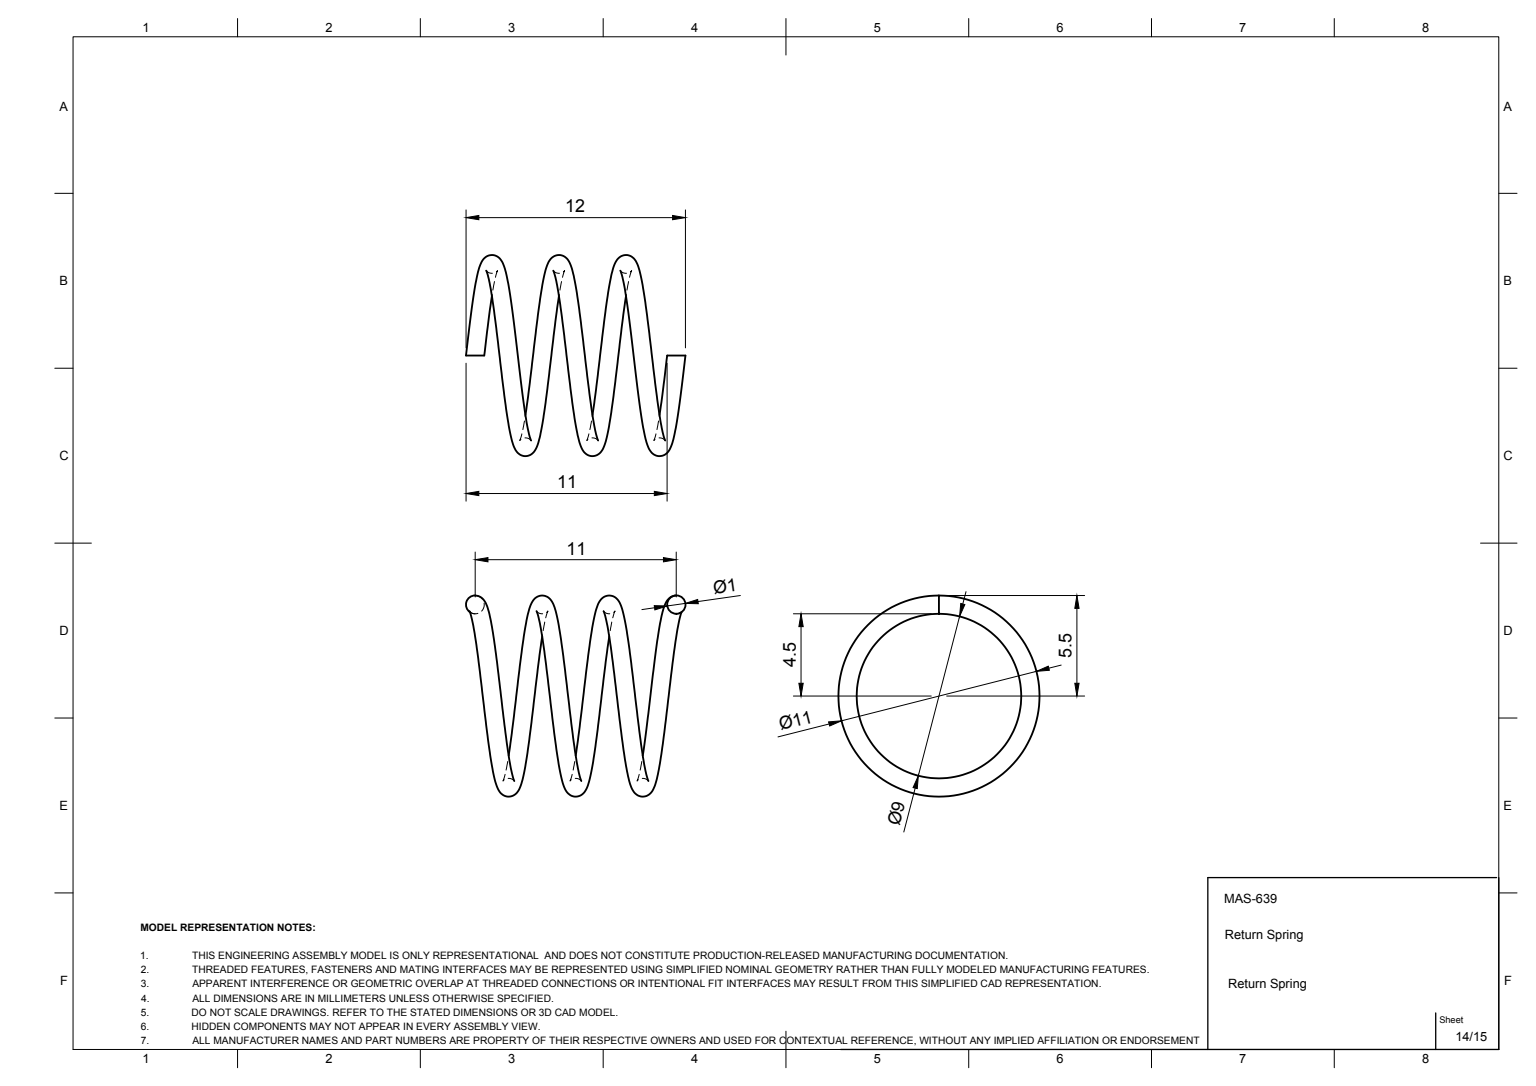
ISO-10303-21;
HEADER;
/* Generated by software containing ST-Developer
 * from STEP Tools, Inc. (www.steptools.com) 
 */

FILE_DESCRIPTION(
/* description */ ('Independent maintained push-to-latch/pull-to-reset mushroom-operator 
CAD. Two opposed spring-loaded ball detents in turned circular seats b
ias both travel stops; direct normally-closed bridge opens6mm when pre
ssed. Rounded palm/pull rim, captured head screw, removable detent clo
sures, native Coil spring families, insulated shared terminals and ord
inary machining features. Manual geometric states and ideal same-mater
ial spring-energy direction only; no electrical/safety certification, 
force/contact dynamics, wear, load or life rating. Requested blue/gray
 visual palette, not safety identification. External wiring/anchors an
d application engineering omitted.'),
/* implementation_level */ '2;1');

FILE_NAME(
/* name */ 'Return spring.step',
/* time_stamp */ '2026-11-08T17:54:26-08:00',
/* author */ (''),
/* organization */ (''),
/* preprocessor_version */ 'ST-DEVELOPER v20.2',
/* originating_system */ 'Autodesk Translation Framework v15.17.0.0',
/* authorisation */ '');

FILE_SCHEMA (('AUTOMOTIVE_DESIGN { 1 0 10303 214 3 1 1 }'));
ENDSEC;

DATA;
#10=MECHANICAL_DESIGN_GEOMETRIC_PRESENTATION_REPRESENTATION('',(#196),#43980);
#162=SHAPE_REPRESENTATION_RELATIONSHIP('SRR','None',#44062,#179);
#179=ADVANCED_BREP_SHAPE_REPRESENTATION('',(#213),#43969);
#196=STYLED_ITEM('',(#44155),#213);
#213=MANIFOLD_SOLID_BREP('Body1',#11237);
#242=B_SPLINE_SURFACE_WITH_KNOTS('',3,3,((#29398,#29399,#29400,#29401,#29402,
#29403,#29404,#29405,#29406,#29407,#29408,#29409,#29410,#29411,#29412,#29413,
#29414,#29415,#29416,#29417,#29418,#29419,#29420,#29421,#29422,#29423,#29424,
#29425,#29426,#29427,#29428,#29429,#29430,#29431,#29432,#29433,#29434,#29435,
#29436,#29437,#29438),(#29439,#29440,#29441,#29442,#29443,#29444,#29445,
#29446,#29447,#29448,#29449,#29450,#29451,#29452,#29453,#29454,#29455,#29456,
#29457,#29458,#29459,#29460,#29461,#29462,#29463,#29464,#29465,#29466,#29467,
#29468,#29469,#29470,#29471,#29472,#29473,#29474,#29475,#29476,#29477,#29478,
#29479),(#29480,#29481,#29482,#29483,#29484,#29485,#29486,#29487,#29488,
#29489,#29490,#29491,#29492,#29493,#29494,#29495,#29496,#29497,#29498,#29499,
#29500,#29501,#29502,#29503,#29504,#29505,#29506,#29507,#29508,#29509,#29510,
#29511,#29512,#29513,#29514,#29515,#29516,#29517,#29518,#29519,#29520),
(#29521,#29522,#29523,#29524,#29525,#29526,#29527,#29528,#29529,#29530,
#29531,#29532,#29533,#29534,#29535,#29536,#29537,#29538,#29539,#29540,#29541,
#29542,#29543,#29544,#29545,#29546,#29547,#29548,#29549,#29550,#29551,#29552,
#29553,#29554,#29555,#29556,#29557,#29558,#29559,#29560,#29561),(#29562,
#29563,#29564,#29565,#29566,#29567,#29568,#29569,#29570,#29571,#29572,#29573,
#29574,#29575,#29576,#29577,#29578,#29579,#29580,#29581,#29582,#29583,#29584,
#29585,#29586,#29587,#29588,#29589,#29590,#29591,#29592,#29593,#29594,#29595,
#29596,#29597,#29598,#29599,#29600,#29601,#29602),(#29603,#29604,#29605,
#29606,#29607,#29608,#29609,#29610,#29611,#29612,#29613,#29614,#29615,#29616,
#29617,#29618,#29619,#29620,#29621,#29622,#29623,#29624,#29625,#29626,#29627,
#29628,#29629,#29630,#29631,#29632,#29633,#29634,#29635,#29636,#29637,#29638,
#29639,#29640,#29641,#29642,#29643),(#29644,#29645,#29646,#29647,#29648,
#29649,#29650,#29651,#29652,#29653,#29654,#29655,#29656,#29657,#29658,#29659,
#29660,#29661,#29662,#29663,#29664,#29665,#29666,#29667,#29668,#29669,#29670,
#29671,#29672,#29673,#29674,#29675,#29676,#29677,#29678,#29679,#29680,#29681,
#29682,#29683,#29684),(#29685,#29686,#29687,#29688,#29689,#29690,#29691,
#29692,#29693,#29694,#29695,#29696,#29697,#29698,#29699,#29700,#29701,#29702,
#29703,#29704,#29705,#29706,#29707,#29708,#29709,#29710,#29711,#29712,#29713,
#29714,#29715,#29716,#29717,#29718,#29719,#29720,#29721,#29722,#29723,#29724,
#29725),(#29726,#29727,#29728,#29729,#29730,#29731,#29732,#29733,#29734,
#29735,#29736,#29737,#29738,#29739,#29740,#29741,#29742,#29743,#29744,#29745,
#29746,#29747,#29748,#29749,#29750,#29751,#29752,#29753,#29754,#29755,#29756,
#29757,#29758,#29759,#29760,#29761,#29762,#29763,#29764,#29765,#29766),
(#29767,#29768,#29769,#29770,#29771,#29772,#29773,#29774,#29775,#29776,
#29777,#29778,#29779,#29780,#29781,#29782,#29783,#29784,#29785,#29786,#29787,
#29788,#29789,#29790,#29791,#29792,#29793,#29794,#29795,#29796,#29797,#29798,
#29799,#29800,#29801,#29802,#29803,#29804,#29805,#29806,#29807)),
 .UNSPECIFIED.,.T.,.F.,.F.,(4,1,1,1,1,1,1,4),(4,1,1,1,1,1,1,1,1,1,1,1,1,
1,1,1,1,1,1,1,1,1,1,1,1,1,1,1,1,1,1,1,1,1,1,1,1,1,4),(-3.14159265358979,
-2.24399475256414,-1.34639685153848,-0.448798950512828,0.448798950512828,
1.34639685153848,2.24399475256414,3.14159265358979),(0.,0.496040945303652,
0.992081890607303,1.48812283591095,1.98416378121461,2.48020472651826,2.97624567182191,
3.47228661712556,3.96832756242921,4.46436850773286,4.96040945303652,5.45645039834017,
5.95249134364382,6.44853228894747,6.94457323425112,7.44061417955477,7.93665512485842,
8.43269607016208,8.92873701546573,9.42477796076938,9.92081890607303,10.4168598513767,
10.9129007966803,11.408941741984,11.9049826872876,12.4010236325913,12.8970645778949,
13.3931055231986,13.8891464685022,14.3851874138059,14.8812283591095,15.3772693044132,
15.8733102497168,16.3693511950205,16.8653921403242,17.3614330856278,17.8574740309315,
18.3535149762351,18.8495559215388),.UNSPECIFIED.);
#411=PLANE('',#11894);
#412=PLANE('',#11895);
#817=FACE_OUTER_BOUND('',#1496,.T.);
#818=FACE_OUTER_BOUND('',#1497,.T.);
#819=FACE_OUTER_BOUND('',#1498,.T.);
#1496=EDGE_LOOP('',(#8645,#8646,#8647,#8648));
#1497=EDGE_LOOP('',(#8649));
#1498=EDGE_LOOP('',(#8650));
#1934=CIRCLE('',#11892,0.05);
#1935=CIRCLE('',#11893,0.05);
#2421=B_SPLINE_CURVE_WITH_KNOTS('',3,(#29811,#29812,#29813,#29814,#29815,
#29816,#29817,#29818,#29819,#29820,#29821,#29822,#29823,#29824,#29825,#29826,
#29827,#29828,#29829,#29830,#29831,#29832,#29833,#29834,#29835,#29836,#29837,
#29838,#29839,#29840,#29841,#29842,#29843,#29844,#29845,#29846,#29847,#29848,
#29849,#29850,#29851),.UNSPECIFIED.,.F.,.F.,(4,1,1,1,1,1,1,1,1,1,1,1,1,
1,1,1,1,1,1,1,1,1,1,1,1,1,1,1,1,1,1,1,1,1,1,1,1,1,4),(0.,0.496040945303652,
0.992081890607303,1.48812283591095,1.98416378121461,2.48020472651826,2.97624567182191,
3.47228661712556,3.96832756242921,4.46436850773286,4.96040945303652,5.45645039834017,
5.95249134364382,6.44853228894747,6.94457323425112,7.44061417955477,7.93665512485842,
8.43269607016208,8.92873701546573,9.42477796076938,9.92081890607303,10.4168598513767,
10.9129007966803,11.408941741984,11.9049826872876,12.4010236325913,12.8970645778949,
13.3931055231986,13.8891464685022,14.3851874138059,14.8812283591095,15.3772693044132,
15.8733102497168,16.3693511950205,16.8653921403242,17.3614330856278,17.8574740309315,
18.3535149762351,18.8495559215388),.UNSPECIFIED.);
#4686=VERTEX_POINT('',#29808);
#4687=VERTEX_POINT('',#29810);
#6092=EDGE_CURVE('',#4686,#4686,#1934,.T.);
#6093=EDGE_CURVE('',#4686,#4687,#2421,.T.);
#6094=EDGE_CURVE('',#4687,#4687,#1935,.T.);
#8645=ORIENTED_EDGE('',*,*,#6092,.T.);
#8646=ORIENTED_EDGE('',*,*,#6093,.T.);
#8647=ORIENTED_EDGE('',*,*,#6094,.F.);
#8648=ORIENTED_EDGE('',*,*,#6093,.F.);
#8649=ORIENTED_EDGE('',*,*,#6094,.T.);
#8650=ORIENTED_EDGE('',*,*,#6092,.F.);
#10942=ADVANCED_FACE('',(#817),#242,.T.);
#10943=ADVANCED_FACE('',(#818),#411,.F.);
#10944=ADVANCED_FACE('',(#819),#412,.T.);
#11237=CLOSED_SHELL('',(#10942,#10943,#10944));
#11891=AXIS2_PLACEMENT_3D('',#29397,#13507,#13508);
#11892=AXIS2_PLACEMENT_3D('',#29809,#13509,#13510);
#11893=AXIS2_PLACEMENT_3D('',#29852,#13511,#13512);
#11894=AXIS2_PLACEMENT_3D('',#29853,#13513,#13514);
#11895=AXIS2_PLACEMENT_3D('',#29854,#13515,#13516);
#13507=DIRECTION('axis',(0.,0.,1.));
#13508=DIRECTION('refdir',(1.,0.,0.));
#13509=DIRECTION('center_axis',(0.,0.,-1.));
#13510=DIRECTION('ref_axis',(-1.,0.,0.));
#13511=DIRECTION('center_axis',(7.34788079488412E-16,0.,-1.));
#13512=DIRECTION('ref_axis',(-1.,0.,-7.34788079488412E-16));
#13513=DIRECTION('center_axis',(-7.34788079488412E-16,0.,1.));
#13514=DIRECTION('ref_axis',(1.,0.,7.34788079488412E-16));
#13515=DIRECTION('center_axis',(0.,0.,1.));
#13516=DIRECTION('ref_axis',(1.,0.,0.));
#29397=CARTESIAN_POINT('',(0.,0.,0.));
#29398=CARTESIAN_POINT('Ctrl Pts',(0.55,-6.12323399573676E-18,0.));
#29399=CARTESIAN_POINT('Ctrl Pts',(0.55,0.00964912280701754,-0.0909408399723361));
#29400=CARTESIAN_POINT('Ctrl Pts',(0.504021197632585,0.0289473684210526,
-0.272733075266705));
#29401=CARTESIAN_POINT('Ctrl Pts',(0.313429112214632,0.0578947368421053,
-0.4797633508545));
#29402=CARTESIAN_POINT('Ctrl Pts',(0.0473287281417178,0.0868421052631579,
-0.571108104224167));
#29403=CARTESIAN_POINT('Ctrl Pts',(-0.230201927212741,0.115789473684211,
-0.52480399893423));
#29404=CARTESIAN_POINT('Ctrl Pts',(-0.452231273974558,0.144736842105263,
-0.351985646771294));
#29405=CARTESIAN_POINT('Ctrl Pts',(-0.565254339124195,0.173684210526316,
-0.0943246722345097));
#29406=CARTESIAN_POINT('Ctrl Pts',(-0.542018875701069,0.202631578947368,
0.186075664943732));
#29407=CARTESIAN_POINT('Ctrl Pts',(-0.388129668188505,0.231578947368421,
0.421620932468086));
#29408=CARTESIAN_POINT('Ctrl Pts',(-0.140680214568305,0.260526315789474,
0.555533945989301));
#29409=CARTESIAN_POINT('Ctrl Pts',(0.140680250766997,0.289473684210526,
0.555533855939788));
#29410=CARTESIAN_POINT('Ctrl Pts',(0.388129540647023,0.318421052631579,
0.421621069647034));
#29411=CARTESIAN_POINT('Ctrl Pts',(0.542019161337126,0.347368421052632,
0.186075408839635));
#29412=CARTESIAN_POINT('Ctrl Pts',(0.565253745898005,0.376315789473684,
-0.0943241631669167));
#29413=CARTESIAN_POINT('Ctrl Pts',(0.452232485289668,0.405263157894737,
-0.351986675242114));
#29414=CARTESIAN_POINT('Ctrl Pts',(0.230199463455902,0.43421052631579,-0.524801912662064));
#29415=CARTESIAN_POINT('Ctrl Pts',(-0.0473237183527974,0.463157894736842,
-0.571112341965111));
#29416=CARTESIAN_POINT('Ctrl Pts',(-0.313439397484805,0.492105263157895,
-0.479754713047896));
#29417=CARTESIAN_POINT('Ctrl Pts',(-0.503999728127626,0.521052631578947,
-0.272751013161366));
#29418=CARTESIAN_POINT('Ctrl Pts',(-0.573069664876904,0.55,-2.39751545989516E-16));
#29419=CARTESIAN_POINT('Ctrl Pts',(-0.503999728127627,0.578947368421053,
0.272751013161366));
#29420=CARTESIAN_POINT('Ctrl Pts',(-0.313439397484805,0.607894736842105,
0.479754713047896));
#29421=CARTESIAN_POINT('Ctrl Pts',(-0.0473237183527982,0.636842105263158,
0.571112341965112));
#29422=CARTESIAN_POINT('Ctrl Pts',(0.230199463455903,0.665789473684211,
0.524801912662064));
#29423=CARTESIAN_POINT('Ctrl Pts',(0.452232485289667,0.694736842105263,
0.351986675242114));
#29424=CARTESIAN_POINT('Ctrl Pts',(0.565253745898007,0.723684210526316,
0.0943241631669169));
#29425=CARTESIAN_POINT('Ctrl Pts',(0.542019161337125,0.752631578947369,
-0.186075408839635));
#29426=CARTESIAN_POINT('Ctrl Pts',(0.388129540647024,0.781578947368421,
-0.421621069647034));
#29427=CARTESIAN_POINT('Ctrl Pts',(0.140680250766998,0.810526315789474,
-0.555533855939788));
#29428=CARTESIAN_POINT('Ctrl Pts',(-0.140680214568305,0.839473684210527,
-0.555533945989301));
#29429=CARTESIAN_POINT('Ctrl Pts',(-0.388129668188505,0.868421052631579,
-0.421620932468086));
#29430=CARTESIAN_POINT('Ctrl Pts',(-0.542018875701069,0.897368421052632,
-0.186075664943732));
#29431=CARTESIAN_POINT('Ctrl Pts',(-0.565254339124195,0.926315789473684,
0.0943246722345097));
#29432=CARTESIAN_POINT('Ctrl Pts',(-0.452231273974558,0.955263157894737,
0.351985646771295));
#29433=CARTESIAN_POINT('Ctrl Pts',(-0.23020192721274,0.984210526315789,
0.52480399893423));
#29434=CARTESIAN_POINT('Ctrl Pts',(0.047328728141718,1.01315789473684,0.571108104224167));
#29435=CARTESIAN_POINT('Ctrl Pts',(0.313429112214631,1.04210526315789,0.4797633508545));
#29436=CARTESIAN_POINT('Ctrl Pts',(0.504021197632586,1.07105263157895,0.272733075266706));
#29437=CARTESIAN_POINT('Ctrl Pts',(0.55,1.09035087719298,0.0909408399723365));
#29438=CARTESIAN_POINT('Ctrl Pts',(0.55,1.1,4.04133443718627E-16));
#29439=CARTESIAN_POINT('Ctrl Pts',(0.55,-0.0149599650170943,0.));
#29440=CARTESIAN_POINT('Ctrl Pts',(0.55,-0.0053108422100767,-0.090963337566431));
#29441=CARTESIAN_POINT('Ctrl Pts',(0.504025597995316,0.0139874034039583,
-0.272722100402085));
#29442=CARTESIAN_POINT('Ctrl Pts',(0.313430222123197,0.0429347718250111,
-0.479772059039409));
#29443=CARTESIAN_POINT('Ctrl Pts',(0.0473293473867347,0.0718821402460636,
-0.57110852263267));
#29444=CARTESIAN_POINT('Ctrl Pts',(-0.230203431837132,0.100829508667116,
-0.524808465895466));
#29445=CARTESIAN_POINT('Ctrl Pts',(-0.452233813118511,0.129776877088169,
-0.351986987289247));
#29446=CARTESIAN_POINT('Ctrl Pts',(-0.565257658331638,0.158724245509222,
-0.0943255642817947));
#29447=CARTESIAN_POINT('Ctrl Pts',(-0.54202199880764,0.187671613930274,
0.186076913937926));
#29448=CARTESIAN_POINT('Ctrl Pts',(-0.388131929047426,0.216618982351327,
0.421623293944921));
#29449=CARTESIAN_POINT('Ctrl Pts',(-0.140681025512686,0.245566350772379,
0.555537208898314));
#29450=CARTESIAN_POINT('Ctrl Pts',(0.140681064202504,0.274513719193432,
0.555537057388092));
#29451=CARTESIAN_POINT('Ctrl Pts',(0.388131792728783,0.303461087614485,
0.421623524751422));
#29452=CARTESIAN_POINT('Ctrl Pts',(0.542022304100625,0.332408456035537,
0.186076483037303));
#29453=CARTESIAN_POINT('Ctrl Pts',(0.565257024280752,0.36135582445659,-0.0943247077642448));
#29454=CARTESIAN_POINT('Ctrl Pts',(0.452235107794019,0.390303192877642,
-0.351988717720502));
#29455=CARTESIAN_POINT('Ctrl Pts',(0.230200798529239,0.419250561298696,
-0.524804955578026));
#29456=CARTESIAN_POINT('Ctrl Pts',(-0.0473239928336781,0.448197929719748,
-0.571115654320144));
#29457=CARTESIAN_POINT('Ctrl Pts',(-0.313441215206083,0.477145298140801,
-0.479757495171017));
#29458=CARTESIAN_POINT('Ctrl Pts',(-0.504002650999897,0.506092666561853,
-0.272752594988184));
#29459=CARTESIAN_POINT('Ctrl Pts',(-0.573072988290107,0.535040034982906,
-2.69720489238206E-16));
#29460=CARTESIAN_POINT('Ctrl Pts',(-0.504002650999898,0.563987403403958,
0.272752594988184));
#29461=CARTESIAN_POINT('Ctrl Pts',(-0.313441215206083,0.59293477182501,
0.479757495171017));
#29462=CARTESIAN_POINT('Ctrl Pts',(-0.0473239928336784,0.621882140246064,
0.571115654320144));
#29463=CARTESIAN_POINT('Ctrl Pts',(0.230200798529239,0.650829508667116,
0.524804955578026));
#29464=CARTESIAN_POINT('Ctrl Pts',(0.452235107794019,0.67977687708817,0.351988717720502));
#29465=CARTESIAN_POINT('Ctrl Pts',(0.565257024280752,0.708724245509221,
0.0943247077642448));
#29466=CARTESIAN_POINT('Ctrl Pts',(0.542022304100626,0.737671613930275,
-0.186076483037303));
#29467=CARTESIAN_POINT('Ctrl Pts',(0.388131792728783,0.766618982351327,
-0.421623524751422));
#29468=CARTESIAN_POINT('Ctrl Pts',(0.140681064202504,0.79556635077238,-0.555537057388092));
#29469=CARTESIAN_POINT('Ctrl Pts',(-0.140681025512686,0.824513719193432,
-0.555537208898314));
#29470=CARTESIAN_POINT('Ctrl Pts',(-0.388131929047426,0.853461087614485,
-0.421623293944921));
#29471=CARTESIAN_POINT('Ctrl Pts',(-0.54202199880764,0.882408456035538,
-0.186076913937926));
#29472=CARTESIAN_POINT('Ctrl Pts',(-0.565257658331638,0.911355824456589,
0.094325564281795));
#29473=CARTESIAN_POINT('Ctrl Pts',(-0.452233813118511,0.940303192877643,
0.351986987289247));
#29474=CARTESIAN_POINT('Ctrl Pts',(-0.230203431837132,0.969250561298695,
0.524808465895466));
#29475=CARTESIAN_POINT('Ctrl Pts',(0.0473293473867349,0.998197929719749,
0.57110852263267));
#29476=CARTESIAN_POINT('Ctrl Pts',(0.313430222123197,1.0271452981408,0.47977205903941));
#29477=CARTESIAN_POINT('Ctrl Pts',(0.504025597995316,1.05609266656185,0.272722100402085));
#29478=CARTESIAN_POINT('Ctrl Pts',(0.55,1.07539091217589,0.0909633375664313));
#29479=CARTESIAN_POINT('Ctrl Pts',(0.55,1.08504003498291,4.04133443718627E-16));
#29480=CARTESIAN_POINT('Ctrl Pts',(0.53570113931992,-0.0447553195607142,
0.));
#29481=CARTESIAN_POINT('Ctrl Pts',(0.53570113931992,-0.0351061967536967,
-0.0885671891766316));
#29482=CARTESIAN_POINT('Ctrl Pts',(0.490915856431254,-0.0158079511396616,
-0.265647154764381));
#29483=CARTESIAN_POINT('Ctrl Pts',(0.305280141935785,0.013139417281391,
-0.467286867853663));
#29484=CARTESIAN_POINT('Ctrl Pts',(0.0460980211403113,0.0420867857024435,
-0.556260302160471));
#29485=CARTESIAN_POINT('Ctrl Pts',(-0.224216526816036,0.0710341541234964,
-0.511158320191165));
#29486=CARTESIAN_POINT('Ctrl Pts',(-0.440473139290293,0.0999815225445487,
-0.342834190341978));
#29487=CARTESIAN_POINT('Ctrl Pts',(-0.550557513729943,0.128928890965602,
-0.0918720543302183));
#29488=CARTESIAN_POINT('Ctrl Pts',(-0.527926205961598,0.157876259386654,
0.181237562509432));
#29489=CARTESIAN_POINT('Ctrl Pts',(-0.378038158462228,0.186823627807707,
0.410658677308307));
#29490=CARTESIAN_POINT('Ctrl Pts',(-0.137022482393337,0.215770996228759,
0.541089854146894));
#29491=CARTESIAN_POINT('Ctrl Pts',(0.1370225166126,0.244718364649812,0.54108979205624));
#29492=CARTESIAN_POINT('Ctrl Pts',(0.378038037895015,0.273665733070865,
0.410658771895499));
#29493=CARTESIAN_POINT('Ctrl Pts',(0.527926475978401,0.302613101491917,
0.181237385921362));
#29494=CARTESIAN_POINT('Ctrl Pts',(0.550556952942761,0.331560469912971,
-0.0918717033197569));
#29495=CARTESIAN_POINT('Ctrl Pts',(0.440474284367836,0.360507838334022,
-0.342834899486897));
#29496=CARTESIAN_POINT('Ctrl Pts',(0.224214197783231,0.389455206755076,
-0.511156881721493));
#29497=CARTESIAN_POINT('Ctrl Pts',(-0.0460932852984628,0.418402575176128,
-0.556263223487983));
#29498=CARTESIAN_POINT('Ctrl Pts',(-0.30528986478313,0.44734994359718,-0.46728092468486));
#29499=CARTESIAN_POINT('Ctrl Pts',(-0.490895560929454,0.476297312018233,
-0.265659392490889));
#29500=CARTESIAN_POINT('Ctrl Pts',(-0.558169655449433,0.505244680439286,
-2.99689432486895E-17));
#29501=CARTESIAN_POINT('Ctrl Pts',(-0.490895560929455,0.534192048860338,
0.265659392490888));
#29502=CARTESIAN_POINT('Ctrl Pts',(-0.305289864783131,0.563139417281392,
0.467280924684859));
#29503=CARTESIAN_POINT('Ctrl Pts',(-0.0460932852984632,0.592086785702444,
0.556263223487983));
#29504=CARTESIAN_POINT('Ctrl Pts',(0.224214197783231,0.621034154123497,
0.511156881721493));
#29505=CARTESIAN_POINT('Ctrl Pts',(0.440474284367836,0.649981522544549,
0.342834899486896));
#29506=CARTESIAN_POINT('Ctrl Pts',(0.550556952942761,0.678928890965602,
0.091871703319757));
#29507=CARTESIAN_POINT('Ctrl Pts',(0.527926475978402,0.707876259386654,
-0.181237385921362));
#29508=CARTESIAN_POINT('Ctrl Pts',(0.378038037895015,0.736823627807706,
-0.410658771895499));
#29509=CARTESIAN_POINT('Ctrl Pts',(0.1370225166126,0.76577099622876,-0.54108979205624));
#29510=CARTESIAN_POINT('Ctrl Pts',(-0.137022482393337,0.794718364649812,
-0.541089854146894));
#29511=CARTESIAN_POINT('Ctrl Pts',(-0.378038158462228,0.823665733070864,
-0.410658677308307));
#29512=CARTESIAN_POINT('Ctrl Pts',(-0.527926205961598,0.852613101491918,
-0.181237562509432));
#29513=CARTESIAN_POINT('Ctrl Pts',(-0.550557513729943,0.88156046991297,
0.0918720543302184));
#29514=CARTESIAN_POINT('Ctrl Pts',(-0.440473139290294,0.910507838334022,
0.342834190341979));
#29515=CARTESIAN_POINT('Ctrl Pts',(-0.224216526816034,0.939455206755075,
0.511158320191165));
#29516=CARTESIAN_POINT('Ctrl Pts',(0.0460980211403112,0.968402575176127,
0.556260302160472));
#29517=CARTESIAN_POINT('Ctrl Pts',(0.305280141935785,0.99734994359718,0.467286867853663));
#29518=CARTESIAN_POINT('Ctrl Pts',(0.490915856431254,1.02629731201823,0.265647154764381));
#29519=CARTESIAN_POINT('Ctrl Pts',(0.53570113931992,1.04559555763227,0.088567189176632));
#29520=CARTESIAN_POINT('Ctrl Pts',(0.53570113931992,1.05524468043929,3.93626811340638E-16));
#29521=CARTESIAN_POINT('Ctrl Pts',(0.487277162951485,-0.055780572102217,
0.));
#29522=CARTESIAN_POINT('Ctrl Pts',(0.487277162951485,-0.0461314492951994,
-0.0805709915657102));
#29523=CARTESIAN_POINT('Ctrl Pts',(0.446542084643265,-0.0268332036811644,
-0.241629603004461));
#29524=CARTESIAN_POINT('Ctrl Pts',(0.277685237629778,0.00211416473988834,
-0.425050866224017));
#29525=CARTESIAN_POINT('Ctrl Pts',(0.0419313205272104,0.0310615331609409,
-0.505978088853912));
#29526=CARTESIAN_POINT('Ctrl Pts',(-0.203949428231782,0.0600089015819936,
-0.464954787158114));
#29527=CARTESIAN_POINT('Ctrl Pts',(-0.400658264797364,0.0889562700030461,
-0.311844738436358));
#29528=CARTESIAN_POINT('Ctrl Pts',(-0.50079204861863,0.117903638424099,
-0.0835677899817997));
#29529=CARTESIAN_POINT('Ctrl Pts',(-0.480206382491451,0.146851006845151,
0.164855378621667));
#29530=CARTESIAN_POINT('Ctrl Pts',(-0.343866889053833,0.175798375266204,
0.373538763876965));
#29531=CARTESIAN_POINT('Ctrl Pts',(-0.12463687145299,0.204745743687256,
0.492180180949036));
#29532=CARTESIAN_POINT('Ctrl Pts',(0.124636903654563,0.23369311210831,0.492180097936035));
#29533=CARTESIAN_POINT('Ctrl Pts',(0.343866775595692,0.262640480529362,
0.373538890336684));
#29534=CARTESIAN_POINT('Ctrl Pts',(0.480206636587103,0.291587848950415,
0.164855142529666));
#29535=CARTESIAN_POINT('Ctrl Pts',(0.500791520897454,0.320535217371467,
-0.0835673206929687));
#29536=CARTESIAN_POINT('Ctrl Pts',(0.400659342357064,0.34948258579252,-0.31184568654235));
#29537=CARTESIAN_POINT('Ctrl Pts',(0.203947236527034,0.378429954213572,
-0.464952863901945));
#29538=CARTESIAN_POINT('Ctrl Pts',(-0.0419268639274376,0.407377322634625,
-0.505981995539795));
#29539=CARTESIAN_POINT('Ctrl Pts',(-0.277694387183471,0.436324691055678,
-0.425042901771534));
#29540=CARTESIAN_POINT('Ctrl Pts',(-0.44652298583642,0.465272059476731,
-0.241646155723996));
#29541=CARTESIAN_POINT('Ctrl Pts',(-0.507716102949532,0.494219427897782,
-1.34860244619103E-16));
#29542=CARTESIAN_POINT('Ctrl Pts',(-0.44652298583642,0.523166796318836,
0.241646155723995));
#29543=CARTESIAN_POINT('Ctrl Pts',(-0.277694387183471,0.552114164739888,
0.425042901771534));
#29544=CARTESIAN_POINT('Ctrl Pts',(-0.0419268639274382,0.581061533160941,
0.505981995539795));
#29545=CARTESIAN_POINT('Ctrl Pts',(0.203947236527034,0.610008901581994,
0.464952863901946));
#29546=CARTESIAN_POINT('Ctrl Pts',(0.400659342357062,0.638956270003045,
0.31184568654235));
#29547=CARTESIAN_POINT('Ctrl Pts',(0.500791520897455,0.667903638424099,
0.083567320692969));
#29548=CARTESIAN_POINT('Ctrl Pts',(0.480206636587102,0.696851006845151,
-0.164855142529666));
#29549=CARTESIAN_POINT('Ctrl Pts',(0.343866775595692,0.725798375266205,
-0.373538890336684));
#29550=CARTESIAN_POINT('Ctrl Pts',(0.124636903654563,0.754745743687256,
-0.492180097936035));
#29551=CARTESIAN_POINT('Ctrl Pts',(-0.12463687145299,0.783693112108309,
-0.492180180949036));
#29552=CARTESIAN_POINT('Ctrl Pts',(-0.343866889053832,0.812640480529363,
-0.373538763876965));
#29553=CARTESIAN_POINT('Ctrl Pts',(-0.480206382491451,0.841587848950416,
-0.164855378621666));
#29554=CARTESIAN_POINT('Ctrl Pts',(-0.50079204861863,0.870535217371465,
0.0835677899817997));
#29555=CARTESIAN_POINT('Ctrl Pts',(-0.400658264797365,0.899482585792521,
0.311844738436358));
#29556=CARTESIAN_POINT('Ctrl Pts',(-0.203949428231782,0.928429954213573,
0.464954787158114));
#29557=CARTESIAN_POINT('Ctrl Pts',(0.0419313205272106,0.957377322634626,
0.505978088853912));
#29558=CARTESIAN_POINT('Ctrl Pts',(0.277685237629778,0.986324691055679,
0.425050866224016));
#29559=CARTESIAN_POINT('Ctrl Pts',(0.446542084643265,1.01527205947673,0.241629603004461));
#29560=CARTESIAN_POINT('Ctrl Pts',(0.487277162951485,1.03457030509077,0.0805709915657105));
#29561=CARTESIAN_POINT('Ctrl Pts',(0.487277162951485,1.04421942789778,3.58045450743683E-16));
#29562=CARTESIAN_POINT('Ctrl Pts',(0.448387246880286,-0.0248419023856354,
0.));
#29563=CARTESIAN_POINT('Ctrl Pts',(0.448387246880286,-0.0151927795786178,
-0.07414422645298));
#29564=CARTESIAN_POINT('Ctrl Pts',(0.410903978185472,0.0041054660354173,
-0.222343197653867));
#29565=CARTESIAN_POINT('Ctrl Pts',(0.255523173753345,0.0330528344564699,
-0.391128689006159));
#29566=CARTESIAN_POINT('Ctrl Pts',(0.038584854538714,0.0620002028775224,
-0.465595707447286));
#29567=CARTESIAN_POINT('Ctrl Pts',(-0.187672332794983,0.0909475712985754,
-0.427847161438827));
#29568=CARTESIAN_POINT('Ctrl Pts',(-0.368681873914515,0.119894939719628,
-0.286956419480487));
#29569=CARTESIAN_POINT('Ctrl Pts',(-0.460824040408845,0.14884230814068,
-0.0768983339117788));
#29570=CARTESIAN_POINT('Ctrl Pts',(-0.44188129815593,0.177789676561733,
0.15169836383255));
#29571=CARTESIAN_POINT('Ctrl Pts',(-0.316423010561111,0.206737044982786,
0.343726769588972));
#29572=CARTESIAN_POINT('Ctrl Pts',(-0.114689651347553,0.235684413403838,
0.452899482496333));
#29573=CARTESIAN_POINT('Ctrl Pts',(0.114689681384317,0.264631781824891,
0.45289939611113));
#29574=CARTESIAN_POINT('Ctrl Pts',(0.316422904730401,0.293579150245943,
0.343726901185811));
#29575=CARTESIAN_POINT('Ctrl Pts',(0.441881535169538,0.322526518666996,
0.151698118149882));
#29576=CARTESIAN_POINT('Ctrl Pts',(0.460823548164688,0.351473887088049,
-0.0768978455591534));
#29577=CARTESIAN_POINT('Ctrl Pts',(0.368682879033298,0.380421255509101,
-0.286957406102108));
#29578=CARTESIAN_POINT('Ctrl Pts',(0.187670288431583,0.409368623930155,
-0.427845160036274));
#29579=CARTESIAN_POINT('Ctrl Pts',(-0.0385806975419882,0.438315992351207,
-0.465599773082623));
#29580=CARTESIAN_POINT('Ctrl Pts',(-0.255531708211606,0.467263360772259,
-0.391120396237365));
#29581=CARTESIAN_POINT('Ctrl Pts',(-0.410886163330746,0.496210729193312,
-0.222360471827706));
#29582=CARTESIAN_POINT('Ctrl Pts',(-0.467195482019691,0.525158097614364,
-2.24767074365171E-16));
#29583=CARTESIAN_POINT('Ctrl Pts',(-0.410886163330746,0.554105466035418,
0.222360471827706));
#29584=CARTESIAN_POINT('Ctrl Pts',(-0.255531708211606,0.583052834456469,
0.391120396237364));
#29585=CARTESIAN_POINT('Ctrl Pts',(-0.0385806975419882,0.612000202877523,
0.465599773082623));
#29586=CARTESIAN_POINT('Ctrl Pts',(0.187670288431583,0.640947571298575,
0.427845160036274));
#29587=CARTESIAN_POINT('Ctrl Pts',(0.368682879033298,0.669894939719628,
0.286957406102107));
#29588=CARTESIAN_POINT('Ctrl Pts',(0.460823548164688,0.69884230814068,0.0768978455591535));
#29589=CARTESIAN_POINT('Ctrl Pts',(0.441881535169539,0.727789676561734,
-0.151698118149882));
#29590=CARTESIAN_POINT('Ctrl Pts',(0.316422904730401,0.756737044982785,
-0.34372690118581));
#29591=CARTESIAN_POINT('Ctrl Pts',(0.114689681384317,0.785684413403839,
-0.452899396111131));
#29592=CARTESIAN_POINT('Ctrl Pts',(-0.114689651347553,0.814631781824892,
-0.452899482496332));
#29593=CARTESIAN_POINT('Ctrl Pts',(-0.316423010561111,0.843579150245942,
-0.343726769588972));
#29594=CARTESIAN_POINT('Ctrl Pts',(-0.44188129815593,0.872526518666998,
-0.15169836383255));
#29595=CARTESIAN_POINT('Ctrl Pts',(-0.460824040408845,0.901473887088049,
0.0768983339117786));
#29596=CARTESIAN_POINT('Ctrl Pts',(-0.368681873914516,0.930421255509102,
0.286956419480488));
#29597=CARTESIAN_POINT('Ctrl Pts',(-0.187672332794982,0.959368623930154,
0.427847161438827));
#29598=CARTESIAN_POINT('Ctrl Pts',(0.038584854538714,0.988315992351207,
0.465595707447287));
#29599=CARTESIAN_POINT('Ctrl Pts',(0.255523173753346,1.01726336077226,0.391128689006158));
#29600=CARTESIAN_POINT('Ctrl Pts',(0.410903978185472,1.04621072919331,0.222343197653867));
#29601=CARTESIAN_POINT('Ctrl Pts',(0.448387246880286,1.06550897480735,0.0741442264529802));
#29602=CARTESIAN_POINT('Ctrl Pts',(0.448387246880286,1.07515809761436,3.29469604002262E-16));
#29603=CARTESIAN_POINT('Ctrl Pts',(0.44846989161077,0.0248083822941807,
0.));
#29604=CARTESIAN_POINT('Ctrl Pts',(0.44846989161077,0.0344575051011982,
-0.0741467389671334));
#29605=CARTESIAN_POINT('Ctrl Pts',(0.410977532641741,0.0537557507152332,
-0.22238961986095));
#29606=CARTESIAN_POINT('Ctrl Pts',(0.255569720392287,0.082703119136286,
-0.391196462921687));
#29607=CARTESIAN_POINT('Ctrl Pts',(0.0385916593292064,0.111650487557339,
-0.465681316533805));
#29608=CARTESIAN_POINT('Ctrl Pts',(-0.187706177786097,0.140597855978391,
-0.427923805769893));
#29609=CARTESIAN_POINT('Ctrl Pts',(-0.368748568900195,0.169545224399444,
-0.287008645427576));
#29610=CARTESIAN_POINT('Ctrl Pts',(-0.460907331901607,0.198492592820497,
-0.0769120652267277));
#29611=CARTESIAN_POINT('Ctrl Pts',(-0.441961195426282,0.227439961241549,
0.151725704994062));
#29612=CARTESIAN_POINT('Ctrl Pts',(-0.316480211389712,0.256387329662602,
0.343788953041849));
#29613=CARTESIAN_POINT('Ctrl Pts',(-0.114710388396602,0.285334698083654,
0.452981341280585));
#29614=CARTESIAN_POINT('Ctrl Pts',(0.1147104172039,0.314282066504708,0.45298128534925));
#29615=CARTESIAN_POINT('Ctrl Pts',(0.316480109890866,0.343229434925759,
0.343789038246103));
#29616=CARTESIAN_POINT('Ctrl Pts',(0.441961422738447,0.372176803346812,
0.151725545923318));
#29617=CARTESIAN_POINT('Ctrl Pts',(0.460906859805993,0.401124171767864,
-0.0769117490360455));
#29618=CARTESIAN_POINT('Ctrl Pts',(0.368749532877446,0.430071540188918,
-0.287009284226811));
#29619=CARTESIAN_POINT('Ctrl Pts',(0.1877042171026,0.45901890860997,-0.427922509983804));
#29620=CARTESIAN_POINT('Ctrl Pts',(-0.0385876724867117,0.487966277031022,
-0.46568394821421));
#29621=CARTESIAN_POINT('Ctrl Pts',(-0.255577905518018,0.516913645452076,
-0.391191106531583));
#29622=CARTESIAN_POINT('Ctrl Pts',(-0.410960446984824,0.545861013873128,
-0.222400672107441));
#29623=CARTESIAN_POINT('Ctrl Pts',(-0.467279945783006,0.57480838229418,
-2.99689432486895E-16));
#29624=CARTESIAN_POINT('Ctrl Pts',(-0.410960446984824,0.603755750715233,
0.222400672107441));
#29625=CARTESIAN_POINT('Ctrl Pts',(-0.255577905518018,0.632703119136285,
0.391191106531583));
#29626=CARTESIAN_POINT('Ctrl Pts',(-0.0385876724867119,0.661650487557339,
0.46568394821421));
#29627=CARTESIAN_POINT('Ctrl Pts',(0.1877042171026,0.690597855978391,0.427922509983805));
#29628=CARTESIAN_POINT('Ctrl Pts',(0.368749532877446,0.719545224399444,
0.287009284226811));
#29629=CARTESIAN_POINT('Ctrl Pts',(0.460906859805992,0.748492592820496,
0.0769117490360456));
#29630=CARTESIAN_POINT('Ctrl Pts',(0.441961422738447,0.777439961241549,
-0.151725545923318));
#29631=CARTESIAN_POINT('Ctrl Pts',(0.316480109890866,0.806387329662602,
-0.343789038246102));
#29632=CARTESIAN_POINT('Ctrl Pts',(0.114710417203901,0.835334698083655,
-0.45298128534925));
#29633=CARTESIAN_POINT('Ctrl Pts',(-0.114710388396602,0.864282066504706,
-0.452981341280585));
#29634=CARTESIAN_POINT('Ctrl Pts',(-0.316480211389712,0.89322943492576,
-0.343788953041849));
#29635=CARTESIAN_POINT('Ctrl Pts',(-0.441961195426283,0.922176803346812,
-0.151725704994062));
#29636=CARTESIAN_POINT('Ctrl Pts',(-0.460907331901607,0.951124171767863,
0.0769120652267278));
#29637=CARTESIAN_POINT('Ctrl Pts',(-0.368748568900195,0.980071540188918,
0.287008645427576));
#29638=CARTESIAN_POINT('Ctrl Pts',(-0.187706177786096,1.00901890860997,
0.427923805769892));
#29639=CARTESIAN_POINT('Ctrl Pts',(0.0385916593292065,1.03796627703102,
0.465681316533805));
#29640=CARTESIAN_POINT('Ctrl Pts',(0.255569720392286,1.06691364545207,0.391196462921687));
#29641=CARTESIAN_POINT('Ctrl Pts',(0.410977532641741,1.09586101387313,0.222389619860949));
#29642=CARTESIAN_POINT('Ctrl Pts',(0.44846989161077,1.11515925948716,0.0741467389671337));
#29643=CARTESIAN_POINT('Ctrl Pts',(0.44846989161077,1.12480838229418,3.29530330365054E-16));
#29644=CARTESIAN_POINT('Ctrl Pts',(0.487239979171329,0.0558629369918963,
0.));
#29645=CARTESIAN_POINT('Ctrl Pts',(0.487239979171329,0.0655120597989138,
-0.0805720968838106));
#29646=CARTESIAN_POINT('Ctrl Pts',(0.446509428085615,0.084810305412949,
-0.241607625921821));
#29647=CARTESIAN_POINT('Ctrl Pts',(0.277664405517879,0.113757673834002,
-0.425021238566598));
#29648=CARTESIAN_POINT('Ctrl Pts',(0.0419283204332873,0.142705042255054,
-0.50593961292168));
#29649=CARTESIAN_POINT('Ctrl Pts',(-0.2039343501116,0.171652410676107,-0.46492074701256));
#29650=CARTESIAN_POINT('Ctrl Pts',(-0.400628509511133,0.200599779097159,
-0.311821373989466));
#29651=CARTESIAN_POINT('Ctrl Pts',(-0.500754903699936,0.229547147518212,
-0.0835617005943787));
#29652=CARTESIAN_POINT('Ctrl Pts',(-0.480170745224076,0.258494515939265,
0.164843201321287));
#29653=CARTESIAN_POINT('Ctrl Pts',(-0.343841377753676,0.287441884360317,
0.373511020777802));
#29654=CARTESIAN_POINT('Ctrl Pts',(-0.124627621963577,0.31638925278137,
0.492143675044313));
#29655=CARTESIAN_POINT('Ctrl Pts',(0.124627654965877,0.345336621202422,
0.492143572221594));
#29656=CARTESIAN_POINT('Ctrl Pts',(0.343841261474276,0.374283989623475,
0.373511177415101));
#29657=CARTESIAN_POINT('Ctrl Pts',(0.480171005638091,0.403231358044527,
0.164842908889717));
#29658=CARTESIAN_POINT('Ctrl Pts',(0.500754362856404,0.432178726465581,
-0.0835611193171623));
#29659=CARTESIAN_POINT('Ctrl Pts',(0.400629613865516,0.461126094886633,
-0.311822548347942));
#29660=CARTESIAN_POINT('Ctrl Pts',(0.203932103907749,0.490073463307686,
-0.464918364765013));
#29661=CARTESIAN_POINT('Ctrl Pts',(-0.0419237530153557,0.519020831728739,
-0.505944452370532));
#29662=CARTESIAN_POINT('Ctrl Pts',(-0.27767378258509,0.54796820014979,-0.425011364051589));
#29663=CARTESIAN_POINT('Ctrl Pts',(-0.446489854366344,0.576915568570844,
-0.241628225884321));
#29664=CARTESIAN_POINT('Ctrl Pts',(-0.507678431017099,0.605862936991897,
-2.99689432486895E-16));
#29665=CARTESIAN_POINT('Ctrl Pts',(-0.446489854366344,0.634810305412948,
0.241628225884321));
#29666=CARTESIAN_POINT('Ctrl Pts',(-0.27767378258509,0.663757673834001,
0.425011364051589));
#29667=CARTESIAN_POINT('Ctrl Pts',(-0.041923753015356,0.692705042255054,
0.505944452370533));
#29668=CARTESIAN_POINT('Ctrl Pts',(0.203932103907749,0.721652410676107,
0.464918364765012));
#29669=CARTESIAN_POINT('Ctrl Pts',(0.400629613865516,0.750599779097159,
0.311822548347942));
#29670=CARTESIAN_POINT('Ctrl Pts',(0.500754362856405,0.779547147518212,
0.0835611193171624));
#29671=CARTESIAN_POINT('Ctrl Pts',(0.48017100563809,0.808494515939265,-0.164842908889718));
#29672=CARTESIAN_POINT('Ctrl Pts',(0.343841261474277,0.837441884360317,
-0.3735111774151));
#29673=CARTESIAN_POINT('Ctrl Pts',(0.124627654965877,0.86638925278137,-0.492143572221595));
#29674=CARTESIAN_POINT('Ctrl Pts',(-0.124627621963577,0.895336621202423,
-0.492143675044312));
#29675=CARTESIAN_POINT('Ctrl Pts',(-0.343841377753676,0.924283989623475,
-0.373511020777802));
#29676=CARTESIAN_POINT('Ctrl Pts',(-0.480170745224076,0.953231358044529,
-0.164843201321287));
#29677=CARTESIAN_POINT('Ctrl Pts',(-0.500754903699936,0.98217872646558,
0.0835617005943788));
#29678=CARTESIAN_POINT('Ctrl Pts',(-0.400628509511134,1.01112609488663,
0.311821373989466));
#29679=CARTESIAN_POINT('Ctrl Pts',(-0.203934350111599,1.04007346330769,
0.46492074701256));
#29680=CARTESIAN_POINT('Ctrl Pts',(0.0419283204332873,1.06902083172874,
0.50593961292168));
#29681=CARTESIAN_POINT('Ctrl Pts',(0.277664405517879,1.09796820014979,0.425021238566598));
#29682=CARTESIAN_POINT('Ctrl Pts',(0.446509428085615,1.12691556857084,0.241607625921822));
#29683=CARTESIAN_POINT('Ctrl Pts',(0.487239979171329,1.14621381418488,0.080572096883811));
#29684=CARTESIAN_POINT('Ctrl Pts',(0.487239979171329,1.1558629369919,3.58018128545275E-16));
#29685=CARTESIAN_POINT('Ctrl Pts',(0.535698098014683,0.0446967718358284,
0.));
#29686=CARTESIAN_POINT('Ctrl Pts',(0.535698098014683,0.054345894642846,
-0.0885628977313501));
#29687=CARTESIAN_POINT('Ctrl Pts',(0.49091232835538,0.0736441402568811,
-0.265647494804398));
#29688=CARTESIAN_POINT('Ctrl Pts',(0.305278221876178,0.102591508677934,
-0.467282748481705));
#29689=CARTESIAN_POINT('Ctrl Pts',(0.0460976551488997,0.131538877098987,
-0.556257073675275));
#29690=CARTESIAN_POINT('Ctrl Pts',(-0.224215000503499,0.160486245520039,
-0.511154665978631));
#29691=CARTESIAN_POINT('Ctrl Pts',(-0.440470211021928,0.189433613941092,
-0.342832018243975));
#29692=CARTESIAN_POINT('Ctrl Pts',(-0.550553829122059,0.218380982362144,
-0.0918713825282206));
#29693=CARTESIAN_POINT('Ctrl Pts',(-0.52792268286081,0.247328350783197,
0.181236323247396));
#29694=CARTESIAN_POINT('Ctrl Pts',(-0.378035631515992,0.27627571920425,
0.410655948223274));
#29695=CARTESIAN_POINT('Ctrl Pts',(-0.137021567919262,0.305223087625302,
0.541086232769947));
#29696=CARTESIAN_POINT('Ctrl Pts',(0.137021601718821,0.334170456046355,
0.54108618102972));
#29697=CARTESIAN_POINT('Ctrl Pts',(0.378035512427552,0.363117824467407,
0.410656027042911));
#29698=CARTESIAN_POINT('Ctrl Pts',(0.527922949565824,0.39206519288846,0.181236176096321));
#29699=CARTESIAN_POINT('Ctrl Pts',(0.550553275213,0.421012561309513,-0.0918710900308351));
#29700=CARTESIAN_POINT('Ctrl Pts',(0.440471342054956,0.449959929730565,
-0.3428326091737));
#29701=CARTESIAN_POINT('Ctrl Pts',(0.224212700036564,0.478907298151618,
-0.511153467328439));
#29702=CARTESIAN_POINT('Ctrl Pts',(-0.0460929773927245,0.50785466657267,
-0.556259507641357));
#29703=CARTESIAN_POINT('Ctrl Pts',(-0.305287825471625,0.536802034993724,
-0.467277803304149));
#29704=CARTESIAN_POINT('Ctrl Pts',(-0.490892281780365,0.565749403414775,
-0.265657617896155));
#29705=CARTESIAN_POINT('Ctrl Pts',(-0.55816592691732,0.594696771835828,
-5.39440978476411E-16));
#29706=CARTESIAN_POINT('Ctrl Pts',(-0.490892281780366,0.623644140256882,
0.265657617896155));
#29707=CARTESIAN_POINT('Ctrl Pts',(-0.305287825471625,0.652591508677933,
0.467277803304148));
#29708=CARTESIAN_POINT('Ctrl Pts',(-0.0460929773927249,0.681538877098987,
0.556259507641358));
#29709=CARTESIAN_POINT('Ctrl Pts',(0.224212700036564,0.710486245520039,
0.51115346732844));
#29710=CARTESIAN_POINT('Ctrl Pts',(0.440471342054955,0.739433613941091,
0.342832609173699));
#29711=CARTESIAN_POINT('Ctrl Pts',(0.550553275213,0.768380982362144,0.0918710900308353));
#29712=CARTESIAN_POINT('Ctrl Pts',(0.527922949565824,0.797328350783197,
-0.181236176096321));
#29713=CARTESIAN_POINT('Ctrl Pts',(0.378035512427552,0.82627571920425,-0.410656027042911));
#29714=CARTESIAN_POINT('Ctrl Pts',(0.137021601718821,0.855223087625302,
-0.541086181029719));
#29715=CARTESIAN_POINT('Ctrl Pts',(-0.137021567919262,0.884170456046355,
-0.541086232769948));
#29716=CARTESIAN_POINT('Ctrl Pts',(-0.378035631515992,0.913117824467408,
-0.410655948223274));
#29717=CARTESIAN_POINT('Ctrl Pts',(-0.52792268286081,0.942065192888461,
-0.181236323247396));
#29718=CARTESIAN_POINT('Ctrl Pts',(-0.550553829122059,0.971012561309512,
0.091871382528221));
#29719=CARTESIAN_POINT('Ctrl Pts',(-0.440470211021928,0.999959929730566,
0.342832018243975));
#29720=CARTESIAN_POINT('Ctrl Pts',(-0.224215000503498,1.02890729815162,
0.511154665978631));
#29721=CARTESIAN_POINT('Ctrl Pts',(0.0460976551488998,1.05785466657267,
0.556257073675275));
#29722=CARTESIAN_POINT('Ctrl Pts',(0.305278221876177,1.08680203499372,0.467282748481705));
#29723=CARTESIAN_POINT('Ctrl Pts',(0.49091232835538,1.11574940341478,0.265647494804399));
#29724=CARTESIAN_POINT('Ctrl Pts',(0.535698098014682,1.13504764902881,0.0885628977313504));
#29725=CARTESIAN_POINT('Ctrl Pts',(0.535698098014683,1.14469677183583,3.93624576625804E-16));
#29726=CARTESIAN_POINT('Ctrl Pts',(0.55,0.0149599650170943,0.));
#29727=CARTESIAN_POINT('Ctrl Pts',(0.55,0.0246090878241118,-0.0909662710727813));
#29728=CARTESIAN_POINT('Ctrl Pts',(0.504026171767425,0.0439073334381469,
-0.272720669367508));
#29729=CARTESIAN_POINT('Ctrl Pts',(0.313430366846398,0.0728547018591995,
-0.47977319451708));
#29730=CARTESIAN_POINT('Ctrl Pts',(0.0473294281313326,0.101802070280252,
-0.571108577189793));
#29731=CARTESIAN_POINT('Ctrl Pts',(-0.23020362802812,0.130749438701305,
-0.524809048351488));
#29732=CARTESIAN_POINT('Ctrl Pts',(-0.452234144202576,0.159696807122357,
-0.351987162082067));
#29733=CARTESIAN_POINT('Ctrl Pts',(-0.565258091129744,0.18864417554341,
-0.094325680597627));
#29734=CARTESIAN_POINT('Ctrl Pts',(-0.54202240603576,0.217591543964463,
0.18607707679678));
#29735=CARTESIAN_POINT('Ctrl Pts',(-0.388132223845349,0.246538912385515,
0.421623601862615));
#29736=CARTESIAN_POINT('Ctrl Pts',(-0.140681131253348,0.275486280806568,
0.555537634355555));
#29737=CARTESIAN_POINT('Ctrl Pts',(0.140681170267988,0.304433649227621,
0.555537474831348));
#29738=CARTESIAN_POINT('Ctrl Pts',(0.388132086382233,0.333381017648673,
0.4216238448774));
#29739=CARTESIAN_POINT('Ctrl Pts',(0.542022713891853,0.362328386069726,
0.186076623104089));
#29740=CARTESIAN_POINT('Ctrl Pts',(0.565257451755643,0.391275754490779,
-0.0943247787753811));
#29741=CARTESIAN_POINT('Ctrl Pts',(0.452235449747614,0.420223122911831,
-0.35198898404335));
#29742=CARTESIAN_POINT('Ctrl Pts',(0.230200972612125,0.449170491332884,
-0.524805352349932));
#29743=CARTESIAN_POINT('Ctrl Pts',(-0.0473240286237898,0.478117859753936,
-0.57111608622475));
#29744=CARTESIAN_POINT('Ctrl Pts',(-0.313441452222401,0.507065228174989,
-0.479757857937623));
#29745=CARTESIAN_POINT('Ctrl Pts',(-0.504003032119066,0.536012596596042,
-0.272752801245751));
#29746=CARTESIAN_POINT('Ctrl Pts',(-0.573073421636609,0.564959965017094,
-2.99689432486895E-16));
#29747=CARTESIAN_POINT('Ctrl Pts',(-0.504003032119067,0.593907333438147,
0.27275280124575));
#29748=CARTESIAN_POINT('Ctrl Pts',(-0.313441452222401,0.6228547018592,0.479757857937623));
#29749=CARTESIAN_POINT('Ctrl Pts',(-0.0473240286237902,0.651802070280252,
0.57111608622475));
#29750=CARTESIAN_POINT('Ctrl Pts',(0.230200972612125,0.680749438701306,
0.524805352349932));
#29751=CARTESIAN_POINT('Ctrl Pts',(0.452235449747613,0.709696807122357,
0.35198898404335));
#29752=CARTESIAN_POINT('Ctrl Pts',(0.565257451755644,0.73864417554341,0.0943247787753813));
#29753=CARTESIAN_POINT('Ctrl Pts',(0.542022713891852,0.767591543964463,
-0.186076623104089));
#29754=CARTESIAN_POINT('Ctrl Pts',(0.388132086382234,0.796538912385515,
-0.4216238448774));
#29755=CARTESIAN_POINT('Ctrl Pts',(0.140681170267989,0.825486280806568,
-0.555537474831348));
#29756=CARTESIAN_POINT('Ctrl Pts',(-0.140681131253348,0.854433649227621,
-0.555537634355555));
#29757=CARTESIAN_POINT('Ctrl Pts',(-0.388132223845348,0.883381017648673,
-0.421623601862615));
#29758=CARTESIAN_POINT('Ctrl Pts',(-0.542022406035761,0.912328386069727,
-0.18607707679678));
#29759=CARTESIAN_POINT('Ctrl Pts',(-0.565258091129743,0.941275754490777,
0.0943256805976271));
#29760=CARTESIAN_POINT('Ctrl Pts',(-0.452234144202576,0.970223122911832,
0.351987162082068));
#29761=CARTESIAN_POINT('Ctrl Pts',(-0.230203628028119,0.999170491332883,
0.524809048351488));
#29762=CARTESIAN_POINT('Ctrl Pts',(0.0473294281313327,1.02811785975394,
0.571108577189792));
#29763=CARTESIAN_POINT('Ctrl Pts',(0.313430366846398,1.05706522817499,0.47977319451708));
#29764=CARTESIAN_POINT('Ctrl Pts',(0.504026171767425,1.08601259659604,0.272720669367508));
#29765=CARTESIAN_POINT('Ctrl Pts',(0.55,1.10531084221008,0.0909662710727816));
#29766=CARTESIAN_POINT('Ctrl Pts',(0.55,1.11495996501709,4.04133443718627E-16));
#29767=CARTESIAN_POINT('Ctrl Pts',(0.55,6.12323399573676E-18,0.));
#29768=CARTESIAN_POINT('Ctrl Pts',(0.55,0.00964912280701755,-0.0909408399723361));
#29769=CARTESIAN_POINT('Ctrl Pts',(0.504021197632585,0.0289473684210526,
-0.272733075266705));
#29770=CARTESIAN_POINT('Ctrl Pts',(0.313429112214632,0.0578947368421053,
-0.4797633508545));
#29771=CARTESIAN_POINT('Ctrl Pts',(0.0473287281417178,0.0868421052631579,
-0.571108104224167));
#29772=CARTESIAN_POINT('Ctrl Pts',(-0.230201927212741,0.115789473684211,
-0.52480399893423));
#29773=CARTESIAN_POINT('Ctrl Pts',(-0.452231273974558,0.144736842105263,
-0.351985646771294));
#29774=CARTESIAN_POINT('Ctrl Pts',(-0.565254339124195,0.173684210526316,
-0.0943246722345097));
#29775=CARTESIAN_POINT('Ctrl Pts',(-0.542018875701069,0.202631578947368,
0.186075664943732));
#29776=CARTESIAN_POINT('Ctrl Pts',(-0.388129668188505,0.231578947368421,
0.421620932468086));
#29777=CARTESIAN_POINT('Ctrl Pts',(-0.140680214568305,0.260526315789474,
0.555533945989301));
#29778=CARTESIAN_POINT('Ctrl Pts',(0.140680250766997,0.289473684210526,
0.555533855939788));
#29779=CARTESIAN_POINT('Ctrl Pts',(0.388129540647023,0.318421052631579,
0.421621069647034));
#29780=CARTESIAN_POINT('Ctrl Pts',(0.542019161337126,0.347368421052632,
0.186075408839635));
#29781=CARTESIAN_POINT('Ctrl Pts',(0.565253745898005,0.376315789473684,
-0.0943241631669167));
#29782=CARTESIAN_POINT('Ctrl Pts',(0.452232485289668,0.405263157894737,
-0.351986675242114));
#29783=CARTESIAN_POINT('Ctrl Pts',(0.230199463455902,0.43421052631579,-0.524801912662064));
#29784=CARTESIAN_POINT('Ctrl Pts',(-0.0473237183527974,0.463157894736842,
-0.571112341965111));
#29785=CARTESIAN_POINT('Ctrl Pts',(-0.313439397484805,0.492105263157895,
-0.479754713047896));
#29786=CARTESIAN_POINT('Ctrl Pts',(-0.503999728127626,0.521052631578947,
-0.272751013161366));
#29787=CARTESIAN_POINT('Ctrl Pts',(-0.573069664876904,0.55,-2.39751545989516E-16));
#29788=CARTESIAN_POINT('Ctrl Pts',(-0.503999728127627,0.578947368421053,
0.272751013161366));
#29789=CARTESIAN_POINT('Ctrl Pts',(-0.313439397484805,0.607894736842105,
0.479754713047896));
#29790=CARTESIAN_POINT('Ctrl Pts',(-0.0473237183527982,0.636842105263158,
0.571112341965112));
#29791=CARTESIAN_POINT('Ctrl Pts',(0.230199463455903,0.665789473684211,
0.524801912662064));
#29792=CARTESIAN_POINT('Ctrl Pts',(0.452232485289667,0.694736842105263,
0.351986675242114));
#29793=CARTESIAN_POINT('Ctrl Pts',(0.565253745898007,0.723684210526316,
0.0943241631669169));
#29794=CARTESIAN_POINT('Ctrl Pts',(0.542019161337125,0.752631578947369,
-0.186075408839635));
#29795=CARTESIAN_POINT('Ctrl Pts',(0.388129540647024,0.781578947368421,
-0.421621069647034));
#29796=CARTESIAN_POINT('Ctrl Pts',(0.140680250766998,0.810526315789474,
-0.555533855939788));
#29797=CARTESIAN_POINT('Ctrl Pts',(-0.140680214568305,0.839473684210527,
-0.555533945989301));
#29798=CARTESIAN_POINT('Ctrl Pts',(-0.388129668188505,0.868421052631579,
-0.421620932468086));
#29799=CARTESIAN_POINT('Ctrl Pts',(-0.542018875701069,0.897368421052632,
-0.186075664943732));
#29800=CARTESIAN_POINT('Ctrl Pts',(-0.565254339124195,0.926315789473684,
0.0943246722345097));
#29801=CARTESIAN_POINT('Ctrl Pts',(-0.452231273974558,0.955263157894737,
0.351985646771295));
#29802=CARTESIAN_POINT('Ctrl Pts',(-0.23020192721274,0.984210526315789,
0.52480399893423));
#29803=CARTESIAN_POINT('Ctrl Pts',(0.047328728141718,1.01315789473684,0.571108104224167));
#29804=CARTESIAN_POINT('Ctrl Pts',(0.313429112214631,1.04210526315789,0.4797633508545));
#29805=CARTESIAN_POINT('Ctrl Pts',(0.504021197632586,1.07105263157895,0.272733075266706));
#29806=CARTESIAN_POINT('Ctrl Pts',(0.55,1.09035087719298,0.0909408399723365));
#29807=CARTESIAN_POINT('Ctrl Pts',(0.55,1.1,4.04133443718627E-16));
#29808=CARTESIAN_POINT('',(0.55,-6.12323399573676E-18,0.));
#29809=CARTESIAN_POINT('Origin',(0.5,0.,0.));
#29810=CARTESIAN_POINT('',(0.55,1.1,4.04133443718627E-16));
#29811=CARTESIAN_POINT('Ctrl Pts',(0.55,6.12323399573676E-18,0.));
#29812=CARTESIAN_POINT('Ctrl Pts',(0.55,0.00964912280701755,-0.0909408399723361));
#29813=CARTESIAN_POINT('Ctrl Pts',(0.504021197632585,0.0289473684210526,
-0.272733075266705));
#29814=CARTESIAN_POINT('Ctrl Pts',(0.313429112214632,0.0578947368421053,
-0.4797633508545));
#29815=CARTESIAN_POINT('Ctrl Pts',(0.0473287281417178,0.0868421052631579,
-0.571108104224167));
#29816=CARTESIAN_POINT('Ctrl Pts',(-0.230201927212741,0.115789473684211,
-0.52480399893423));
#29817=CARTESIAN_POINT('Ctrl Pts',(-0.452231273974558,0.144736842105263,
-0.351985646771294));
#29818=CARTESIAN_POINT('Ctrl Pts',(-0.565254339124195,0.173684210526316,
-0.0943246722345097));
#29819=CARTESIAN_POINT('Ctrl Pts',(-0.542018875701069,0.202631578947368,
0.186075664943732));
#29820=CARTESIAN_POINT('Ctrl Pts',(-0.388129668188505,0.231578947368421,
0.421620932468086));
#29821=CARTESIAN_POINT('Ctrl Pts',(-0.140680214568305,0.260526315789474,
0.555533945989301));
#29822=CARTESIAN_POINT('Ctrl Pts',(0.140680250766997,0.289473684210526,
0.555533855939788));
#29823=CARTESIAN_POINT('Ctrl Pts',(0.388129540647023,0.318421052631579,
0.421621069647034));
#29824=CARTESIAN_POINT('Ctrl Pts',(0.542019161337126,0.347368421052632,
0.186075408839635));
#29825=CARTESIAN_POINT('Ctrl Pts',(0.565253745898005,0.376315789473684,
-0.0943241631669167));
#29826=CARTESIAN_POINT('Ctrl Pts',(0.452232485289668,0.405263157894737,
-0.351986675242114));
#29827=CARTESIAN_POINT('Ctrl Pts',(0.230199463455902,0.43421052631579,-0.524801912662064));
#29828=CARTESIAN_POINT('Ctrl Pts',(-0.0473237183527974,0.463157894736842,
-0.571112341965111));
#29829=CARTESIAN_POINT('Ctrl Pts',(-0.313439397484805,0.492105263157895,
-0.479754713047896));
#29830=CARTESIAN_POINT('Ctrl Pts',(-0.503999728127626,0.521052631578947,
-0.272751013161366));
#29831=CARTESIAN_POINT('Ctrl Pts',(-0.573069664876904,0.55,-2.39751545989516E-16));
#29832=CARTESIAN_POINT('Ctrl Pts',(-0.503999728127627,0.578947368421053,
0.272751013161366));
#29833=CARTESIAN_POINT('Ctrl Pts',(-0.313439397484805,0.607894736842105,
0.479754713047896));
#29834=CARTESIAN_POINT('Ctrl Pts',(-0.0473237183527982,0.636842105263158,
0.571112341965112));
#29835=CARTESIAN_POINT('Ctrl Pts',(0.230199463455903,0.665789473684211,
0.524801912662064));
#29836=CARTESIAN_POINT('Ctrl Pts',(0.452232485289667,0.694736842105263,
0.351986675242114));
#29837=CARTESIAN_POINT('Ctrl Pts',(0.565253745898007,0.723684210526316,
0.0943241631669169));
#29838=CARTESIAN_POINT('Ctrl Pts',(0.542019161337125,0.752631578947369,
-0.186075408839635));
#29839=CARTESIAN_POINT('Ctrl Pts',(0.388129540647024,0.781578947368421,
-0.421621069647034));
#29840=CARTESIAN_POINT('Ctrl Pts',(0.140680250766998,0.810526315789474,
-0.555533855939788));
#29841=CARTESIAN_POINT('Ctrl Pts',(-0.140680214568305,0.839473684210527,
-0.555533945989301));
#29842=CARTESIAN_POINT('Ctrl Pts',(-0.388129668188505,0.868421052631579,
-0.421620932468086));
#29843=CARTESIAN_POINT('Ctrl Pts',(-0.542018875701069,0.897368421052632,
-0.186075664943732));
#29844=CARTESIAN_POINT('Ctrl Pts',(-0.565254339124195,0.926315789473684,
0.0943246722345097));
#29845=CARTESIAN_POINT('Ctrl Pts',(-0.452231273974558,0.955263157894737,
0.351985646771295));
#29846=CARTESIAN_POINT('Ctrl Pts',(-0.23020192721274,0.984210526315789,
0.52480399893423));
#29847=CARTESIAN_POINT('Ctrl Pts',(0.047328728141718,1.01315789473684,0.571108104224167));
#29848=CARTESIAN_POINT('Ctrl Pts',(0.313429112214631,1.04210526315789,0.4797633508545));
#29849=CARTESIAN_POINT('Ctrl Pts',(0.504021197632586,1.07105263157895,0.272733075266706));
#29850=CARTESIAN_POINT('Ctrl Pts',(0.55,1.09035087719298,0.0909408399723365));
#29851=CARTESIAN_POINT('Ctrl Pts',(0.55,1.1,4.04133443718627E-16));
#29852=CARTESIAN_POINT('Origin',(0.5,1.1,3.67394039744206E-16));
#29853=CARTESIAN_POINT('Origin',(0.5,1.1,3.67394039744206E-16));
#29854=CARTESIAN_POINT('Origin',(0.5,7.2280144832367E-19,0.));
#43950=UNCERTAINTY_MEASURE_WITH_UNIT(LENGTH_MEASURE(0.001),#43981,
'DISTANCE_ACCURACY_VALUE',
'Maximum model space distance between geometric entities at asserted c
onnectivities');
#43961=UNCERTAINTY_MEASURE_WITH_UNIT(LENGTH_MEASURE(0.001),#43981,
'DISTANCE_ACCURACY_VALUE',
'Maximum model space distance between geometric entities at asserted c
onnectivities');
#43969=(
GEOMETRIC_REPRESENTATION_CONTEXT(3)
GLOBAL_UNCERTAINTY_ASSIGNED_CONTEXT((#43950))
GLOBAL_UNIT_ASSIGNED_CONTEXT((#43981,#43983,#43984))
REPRESENTATION_CONTEXT('','3D')
);
#43980=(
GEOMETRIC_REPRESENTATION_CONTEXT(3)
GLOBAL_UNCERTAINTY_ASSIGNED_CONTEXT((#43961))
GLOBAL_UNIT_ASSIGNED_CONTEXT((#43981,#43983,#43984))
REPRESENTATION_CONTEXT('','3D')
);
#43981=(
LENGTH_UNIT()
NAMED_UNIT(*)
SI_UNIT(.CENTI.,.METRE.)
);
#43983=(
NAMED_UNIT(*)
PLANE_ANGLE_UNIT()
SI_UNIT($,.RADIAN.)
);
#43984=(
NAMED_UNIT(*)
SI_UNIT($,.STERADIAN.)
SOLID_ANGLE_UNIT()
);
#43992=SHAPE_DEFINITION_REPRESENTATION(#44010,#44062);
#44010=PRODUCT_DEFINITION_SHAPE('',$,#44081);
#44062=SHAPE_REPRESENTATION('',(#11891),#43969);
#44073=PRODUCT_DEFINITION_CONTEXT('part definition',#44129,'design');
#44081=PRODUCT_DEFINITION('Return Spring','Return spring',#44099,#44073);
#44099=PRODUCT_DEFINITION_FORMATION('',$,#44138);
#44129=APPLICATION_CONTEXT(
'Core Data for Automotive Mechanical Design Process');
#44130=PRODUCT_CONTEXT('part definition',#44129,'mechanical');
#44138=PRODUCT('Return Spring','Return spring',$,(#44130));
#44155=PRESENTATION_STYLE_ASSIGNMENT((#44167));
#44167=SURFACE_STYLE_USAGE(.BOTH.,#44179);
#44179=SURFACE_SIDE_STYLE('',(#44191));
#44191=SURFACE_STYLE_FILL_AREA(#44203);
#44203=FILL_AREA_STYLE('Spring gray',(#44215));
#44215=FILL_AREA_STYLE_COLOUR('Spring gray',#44227);
#44227=COLOUR_RGB('Spring gray',0.407843137254902,0.447058823529412,0.498039215686275);
ENDSEC;
END-ISO-10303-21;
